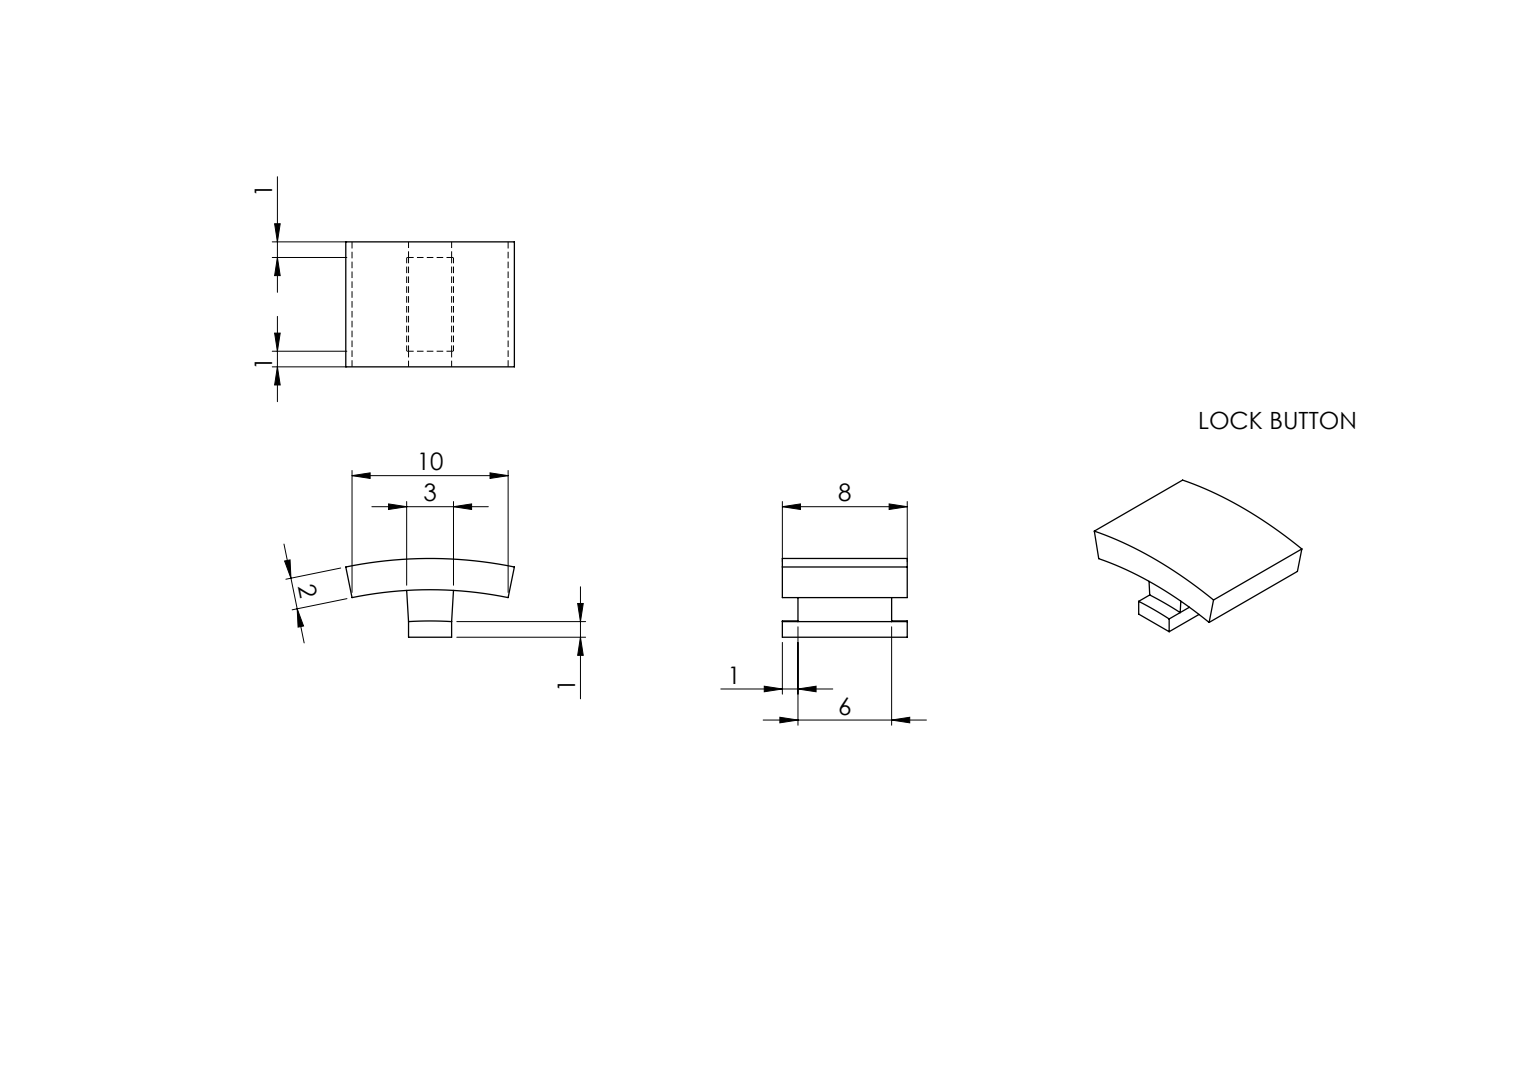
ISO-10303-21;
HEADER;
FILE_DESCRIPTION (('STEP AP214'),
    '1' );
FILE_NAME ('Lock Button.step',
    '2026-10-23T14:45:25',
    ( '' ),
    ( '' ),
    'SwSTEP 2.0',
    'SolidWorks 2026',
    '' );
FILE_SCHEMA (( 'AUTOMOTIVE_DESIGN' ));
ENDSEC;

DATA;
#2=DIRECTION ( 'NONE',  ( -1.000000000000000000, 0.000000000000000000, 0.000000000000000000 ) ) ;
#23=EDGE_CURVE ( 'NONE', #5658, #4842, #4898, .T. ) ;
#26=FILL_AREA_STYLE ('',( #3055 ) ) ;
#34=DIRECTION ( 'NONE',  ( 0.000000000000000000, 0.000000000000000000, -1.000000000000000000 ) ) ;
#40=CIRCLE ( 'NONE', #4910, 25.00000000000000000 ) ;
#55=CARTESIAN_POINT ( 'NONE',  ( 1.380000000000002336, 22.95856267278071172, 12.00000000000000000 ) ) ;
#65=ORIENTED_EDGE ( 'NONE', *, *, #4214, .F. ) ;
#72=VECTOR ( 'NONE', #3186, 1000.000000000000000 ) ;
#83=( NAMED_UNIT ( * ) SI_UNIT ( $, .STERADIAN. ) SOLID_ANGLE_UNIT ( ) );
#84=CARTESIAN_POINT ( 'NONE',  ( 1.380000000000002558, 22.95856267278071527, 1.371299631966804711 ) ) ;
#116=DIRECTION ( 'NONE',  ( 2.385244779468107388E-15, 1.000000000000000000, 0.000000000000000000 ) ) ;
#117=ORIENTED_EDGE ( 'NONE', *, *, #2522, .T. ) ;
#136=PLANE ( 'NONE',  #3174 ) ;
#139=ORIENTED_EDGE ( 'NONE', *, *, #5614, .T. ) ;
#142=LINE ( 'NONE', #1986, #246 ) ;
#143=SHAPE_REPRESENTATION ( 'Lock Button', ( #1336 ), #3242 ) ;
#175=DIRECTION ( 'NONE',  ( -0.000000000000000000, -0.000000000000000000, 1.000000000000000000 ) ) ;
#176=CARTESIAN_POINT ( 'NONE',  ( 1.380000000000002558, 22.95856267278071527, 11.00000000000000000 ) ) ;
#185=FACE_OUTER_BOUND ( 'NONE', #2391, .T. ) ;
#203=LINE ( 'NONE', #3710, #3455 ) ;
#213=DIRECTION ( 'NONE',  ( 0.000000000000000000, 0.000000000000000000, -1.000000000000000000 ) ) ;
#219=AXIS2_PLACEMENT_3D ( 'NONE', #5135, #3840, #5044 ) ;
#220=ORIENTED_EDGE ( 'NONE', *, *, #4170, .T. ) ;
#230=CARTESIAN_POINT ( 'NONE',  ( 1.380000000000002558, 22.95856267278071527, 11.00000000000000000 ) ) ;
#246=VECTOR ( 'NONE', #2299, 1000.000000000000000 ) ;
#267=EDGE_CURVE ( 'NONE', #1755, #5130, #3687, .T. ) ;
#278=FACE_OUTER_BOUND ( 'NONE', #3102, .T. ) ;
#283=CARTESIAN_POINT ( 'NONE',  ( 0.000000000000000000, 0.000000000000000000, 0.000000000000000000 ) ) ;
#295=DIRECTION ( 'NONE',  ( -0.2000000000000000111, 0.9797958971132711969, 0.000000000000000000 ) ) ;
#302=PLANE ( 'NONE',  #1328 ) ;
#303=VECTOR ( 'NONE', #5105, 1000.000000000000000 ) ;
#316=PLANE ( 'NONE',  #4655 ) ;
#324=DIRECTION ( 'NONE',  ( -0.9797958971132711969, 0.2000000000000004552, 0.000000000000000000 ) ) ;
#326=LINE ( 'NONE', #2542, #614 ) ;
#333=ORIENTED_EDGE ( 'NONE', *, *, #340, .F. ) ;
#340=EDGE_CURVE ( 'NONE', #1755, #3088, #1648, .T. ) ;
#346=DIRECTION ( 'NONE',  ( 0.000000000000000000, 0.000000000000000000, -1.000000000000000000 ) ) ;
#357=DIRECTION ( 'NONE',  ( -1.000000000000000000, 0.000000000000000000, 0.000000000000000000 ) ) ;
#364=EDGE_CURVE ( 'NONE', #1139, #4301, #2266, .T. ) ;
#373=DIRECTION ( 'NONE',  ( -0.000000000000000000, -0.000000000000000000, 1.000000000000000000 ) ) ;
#378=DIRECTION ( 'NONE',  ( -0.2000000000000004552, -0.9797958971132711969, 0.000000000000000000 ) ) ;
#389=PRODUCT_DEFINITION_FORMATION_WITH_SPECIFIED_SOURCE ( 'ANY', '', #4589, .NOT_KNOWN. ) ;
#398=ADVANCED_FACE ( 'NONE', ( #2533 ), #316, .T. ) ;
#413=DIRECTION ( 'NONE',  ( 0.000000000000000000, 0.000000000000000000, -1.000000000000000000 ) ) ;
#417=AXIS2_PLACEMENT_3D ( 'NONE', #1217, #3404, #5182 ) ;
#426=AXIS2_PLACEMENT_3D ( 'NONE', #2854, #1529, #4607 ) ;
#431=( NAMED_UNIT ( * ) SI_UNIT ( $, .STERADIAN. ) SOLID_ANGLE_UNIT ( ) );
#435=CARTESIAN_POINT ( 'NONE',  ( 0.000000000000000000, 21.95856267278071527, 4.000000000000000000 ) ) ;
#438=VECTOR ( 'NONE', #2, 1000.000000000000000 ) ;
#465=VERTEX_POINT ( 'NONE', #2969 ) ;
#474=CARTESIAN_POINT ( 'NONE',  ( 1.500000000000003109, 24.95495942693557012, 11.00000000000000000 ) ) ;
#486=DIRECTION ( 'NONE',  ( 1.000000000000000000, -2.385244779468107388E-15, 0.000000000000000000 ) ) ;
#489=CIRCLE ( 'NONE', #219, 25.00000000000000355 ) ;
#491=LINE ( 'NONE', #4006, #5389 ) ;
#496=AXIS2_PLACEMENT_3D ( 'NONE', #3912, #833, #2699 ) ;
#500=EDGE_CURVE ( 'NONE', #1550, #3604, #3484, .T. ) ;
#509=ADVANCED_FACE ( 'NONE', ( #3541 ), #2245, .F. ) ;
#526=DIRECTION ( 'NONE',  ( 1.000000000000000000, 0.000000000000000000, 0.000000000000000000 ) ) ;
#542=DIRECTION ( 'NONE',  ( -1.000000000000000000, 0.000000000000000000, 0.000000000000000000 ) ) ;
#544=ORIENTED_EDGE ( 'NONE', *, *, #3049, .T. ) ;
#546=CARTESIAN_POINT ( 'NONE',  ( -5.399999999999998579, 26.45448922205832787, 12.00000000000000000 ) ) ;
#563=ORIENTED_EDGE ( 'NONE', *, *, #3394, .F. ) ;
#565=FACE_OUTER_BOUND ( 'NONE', #5136, .T. ) ;
#574=CARTESIAN_POINT ( 'NONE',  ( 0.000000000000000000, 0.000000000000000000, 12.00000000000000000 ) ) ;
#575=UNCERTAINTY_MEASURE_WITH_UNIT (LENGTH_MEASURE( 1.000000000000000082E-05 ), #4830, 'distance_accuracy_value', 'NONE');
#607=AXIS2_PLACEMENT_3D ( 'NONE', #2707, #486, #5329 ) ;
#612=VECTOR ( 'NONE', #526, 1000.000000000000000 ) ;
#614=VECTOR ( 'NONE', #4305, 1000.000000000000000 ) ;
#620=PLANE ( 'NONE',  #2643 ) ;
#672=LINE ( 'NONE', #2886, #5086 ) ;
#682=EDGE_LOOP ( 'NONE', ( #5307, #2020, #1568, #4865 ) ) ;
#686=CARTESIAN_POINT ( 'NONE',  ( -4.999999999999998224, 24.49489742783178414, 12.00000000000000000 ) ) ;
#694=ADVANCED_BREP_SHAPE_REPRESENTATION ( '', ( #4492, #1336 ), #3242 ) ;
#709=CARTESIAN_POINT ( 'NONE',  ( 0.000000000000000000, 0.000000000000000000, 11.00000000000000000 ) ) ;
#731=CARTESIAN_POINT ( 'NONE',  ( 5.000000000000001776, 24.49489742783178414, 4.000000000000000000 ) ) ;
#733=DIRECTION ( 'NONE',  ( -1.000000000000000000, 0.000000000000000000, 0.000000000000000000 ) ) ;
#739=ORIENTED_EDGE ( 'NONE', *, *, #1001, .T. ) ;
#748=EDGE_CURVE ( 'NONE', #4516, #5521, #2767, .T. ) ;
#752=EDGE_CURVE ( 'NONE', #5339, #4697, #142, .T. ) ;
#758=CARTESIAN_POINT ( 'NONE',  ( 5.000000000000001776, 24.49489742783178414, 12.00000000000000000 ) ) ;
#759=COLOUR_RGB ( '',0.8941176470588234615, 0.8941176470588234615, 0.8941176470588234615 ) ;
#760=VERTEX_POINT ( 'NONE', #4973 ) ;
#766=ORIENTED_EDGE ( 'NONE', *, *, #23, .T. ) ;
#784=DIRECTION ( 'NONE',  ( -1.000000000000000000, 0.000000000000000000, -0.000000000000000000 ) ) ;
#790=DIRECTION ( 'NONE',  ( -1.000000000000000000, 0.000000000000000000, 0.000000000000000000 ) ) ;
#793=PRODUCT_DEFINITION_CONTEXT ( 'detailed design', #822, 'design' ) ;
#794=VECTOR ( 'NONE', #5528, 1000.000000000000000 ) ;
#798=VECTOR ( 'NONE', #1497, 1000.000000000000114 ) ;
#819=LINE ( 'NONE', #5620, #3283 ) ;
#822=APPLICATION_CONTEXT ( 'automotive_design' ) ;
#833=DIRECTION ( 'NONE',  ( 0.000000000000000000, 0.000000000000000000, -1.000000000000000000 ) ) ;
#841=VERTEX_POINT ( 'NONE', #4160 ) ;
#847=DIRECTION ( 'NONE',  ( -1.000000000000000000, 0.000000000000000000, -0.000000000000000000 ) ) ;
#855=PRODUCT_CONTEXT ( 'NONE', #5414, 'mechanical' ) ;
#880=ORIENTED_EDGE ( 'NONE', *, *, #4681, .T. ) ;
#884=SHAPE_DEFINITION_REPRESENTATION ( #3763, #143 ) ;
#918=( NAMED_UNIT ( * ) PLANE_ANGLE_UNIT ( ) SI_UNIT ( $, .RADIAN. ) );
#946=( LENGTH_UNIT ( ) NAMED_UNIT ( * ) SI_UNIT ( .MILLI., .METRE. ) );
#955=DIRECTION ( 'NONE',  ( -0.000000000000000000, -0.000000000000000000, 1.000000000000000000 ) ) ;
#957=CARTESIAN_POINT ( 'NONE',  ( 0.000000000000000000, 21.95856267278071527, 12.00000000000000000 ) ) ;
#960=VECTOR ( 'NONE', #1765, 999.9999999999998863 ) ;
#977=CIRCLE ( 'NONE', #3188, 23.00000000000000000 ) ;
#980=PLANE ( 'NONE',  #3743 ) ;
#982=DIRECTION ( 'NONE',  ( 0.000000000000000000, 0.000000000000000000, -1.000000000000000000 ) ) ;
#984=VECTOR ( 'NONE', #3012, 1000.000000000000000 ) ;
#1001=EDGE_CURVE ( 'NONE', #4842, #1005, #1915, .T. ) ;
#1005=VERTEX_POINT ( 'NONE', #2808 ) ;
#1008=ADVANCED_FACE ( 'NONE', ( #4558 ), #620, .T. ) ;
#1034=CYLINDRICAL_SURFACE ( 'NONE', #426, 23.00000000000000000 ) ;
#1045=DIRECTION ( 'NONE',  ( 0.000000000000000000, 0.000000000000000000, -1.000000000000000000 ) ) ;
#1051=ORIENTED_EDGE ( 'NONE', *, *, #3485, .T. ) ;
#1055=CARTESIAN_POINT ( 'NONE',  ( 0.000000000000000000, 0.000000000000000000, 15.94994774640597512 ) ) ;
#1065=DIRECTION ( 'NONE',  ( -1.000000000000000000, 0.000000000000000000, 0.000000000000000000 ) ) ;
#1068=ORIENTED_EDGE ( 'NONE', *, *, #1175, .F. ) ;
#1083=EDGE_CURVE ( 'NONE', #3693, #5521, #326, .T. ) ;
#1097=ORIENTED_EDGE ( 'NONE', *, *, #1110, .F. ) ;
#1110=EDGE_CURVE ( 'NONE', #3088, #5521, #1262, .T. ) ;
#1123=CARTESIAN_POINT ( 'NONE',  ( -5.399999999999998579, 26.45448922205832787, 4.000000000000000000 ) ) ;
#1139=VERTEX_POINT ( 'NONE', #5568 ) ;
#1152=AXIS2_PLACEMENT_3D ( 'NONE', #4637, #2913, #3802 ) ;
#1157=DIRECTION ( 'NONE',  ( 1.000000000000000000, 0.000000000000000000, 0.000000000000000000 ) ) ;
#1160=EDGE_CURVE ( 'NONE', #3604, #1139, #819, .T. ) ;
#1175=EDGE_CURVE ( 'NONE', #3721, #1005, #1198, .T. ) ;
#1187=ORIENTED_EDGE ( 'NONE', *, *, #3561, .T. ) ;
#1198=LINE ( 'NONE', #1680, #984 ) ;
#1203=EDGE_CURVE ( 'NONE', #4044, #4516, #2600, .T. ) ;
#1217=CARTESIAN_POINT ( 'NONE',  ( 0.000000000000000000, 0.000000000000000000, 24.08672805191341482 ) ) ;
#1228=ORIENTED_EDGE ( 'NONE', *, *, #2292, .F. ) ;
#1235=CIRCLE ( 'NONE', #5096, 23.00000000000000000 ) ;
#1245=EDGE_CURVE ( 'NONE', #5361, #1550, #5253, .T. ) ;
#1246=PLANE ( 'NONE',  #4536 ) ;
#1262=CIRCLE ( 'NONE', #1808, 25.00000000000000000 ) ;
#1277=ADVANCED_FACE ( 'NONE', ( #4801 ), #980, .F. ) ;
#1290=ORIENTED_EDGE ( 'NONE', *, *, #4170, .F. ) ;
#1306=CARTESIAN_POINT ( 'NONE',  ( -1.500000000000000888, 24.95495942693557012, 11.00000000000000000 ) ) ;
#1308=CARTESIAN_POINT ( 'NONE',  ( -5.399999999999998579, 26.45448922205832787, 12.00000000000000000 ) ) ;
#1319=ORIENTED_EDGE ( 'NONE', *, *, #1160, .F. ) ;
#1321=AXIS2_PLACEMENT_3D ( 'NONE', #84, #4799, #4376 ) ;
#1328=AXIS2_PLACEMENT_3D ( 'NONE', #2036, #2064, #3821 ) ;
#1336=AXIS2_PLACEMENT_3D ( 'NONE', #283, #2997, #5213 ) ;
#1374=ORIENTED_EDGE ( 'NONE', *, *, #340, .T. ) ;
#1382=LINE ( 'NONE', #1649, #3536 ) ;
#1392=ORIENTED_EDGE ( 'NONE', *, *, #2121, .T. ) ;
#1405=EDGE_CURVE ( 'NONE', #1005, #3984, #4403, .T. ) ;
#1408=PLANE ( 'NONE',  #1321 ) ;
#1468=ORIENTED_EDGE ( 'NONE', *, *, #752, .T. ) ;
#1487=DIRECTION ( 'NONE',  ( -1.000000000000000000, 0.000000000000000000, 0.000000000000000000 ) ) ;
#1495=FACE_OUTER_BOUND ( 'NONE', #3746, .T. ) ;
#1496=VERTEX_POINT ( 'NONE', #2353 ) ;
#1497=DIRECTION ( 'NONE',  ( 0.06000000000000008105, -0.9981983770774224274, 0.000000000000000000 ) ) ;
#1504=ORIENTED_EDGE ( 'NONE', *, *, #4283, .F. ) ;
#1513=ORIENTED_EDGE ( 'NONE', *, *, #5599, .T. ) ;
#1515=CIRCLE ( 'NONE', #1152, 23.00000000000000000 ) ;
#1527=CARTESIAN_POINT ( 'NONE',  ( -1.380000000000002558, 21.95856267278071527, 12.00000000000000000 ) ) ;
#1529=DIRECTION ( 'NONE',  ( 0.000000000000000000, 0.000000000000000000, -1.000000000000000000 ) ) ;
#1535=CLOSED_SHELL ( 'NONE', ( #2866, #5174, #4061, #4351, #5113, #4620, #3495, #398, #2220, #509, #5195, #4989, #1008, #3147, #1277, #2437, #5438 ) ) ;
#1539=DIRECTION ( 'NONE',  ( 0.000000000000000000, 0.000000000000000000, -1.000000000000000000 ) ) ;
#1550=VERTEX_POINT ( 'NONE', #546 ) ;
#1559=CARTESIAN_POINT ( 'NONE',  ( 1.380000000000002336, 22.95856267278071172, 15.94994774640597512 ) ) ;
#1568=ORIENTED_EDGE ( 'NONE', *, *, #4598, .T. ) ;
#1586=ORIENTED_EDGE ( 'NONE', *, *, #364, .F. ) ;
#1602=ORIENTED_EDGE ( 'NONE', *, *, #2842, .F. ) ;
#1613=VECTOR ( 'NONE', #378, 999.9999999999998863 ) ;
#1626=LINE ( 'NONE', #758, #1613 ) ;
#1634=EDGE_LOOP ( 'NONE', ( #1374, #3177, #5626, #5423 ) ) ;
#1648=LINE ( 'NONE', #4324, #4111 ) ;
#1649=CARTESIAN_POINT ( 'NONE',  ( 1.380000000000002558, 22.95856267278071527, 5.000000000000000000 ) ) ;
#1672=ORIENTED_EDGE ( 'NONE', *, *, #2121, .F. ) ;
#1680=CARTESIAN_POINT ( 'NONE',  ( 1.380000000000002558, 0.000000000000000000, 4.000000000000000000 ) ) ;
#1702=FACE_OUTER_BOUND ( 'NONE', #3953, .T. ) ;
#1711=DIRECTION ( 'NONE',  ( 0.000000000000000000, 0.000000000000000000, -1.000000000000000000 ) ) ;
#1728=FACE_OUTER_BOUND ( 'NONE', #4142, .T. ) ;
#1738=EDGE_LOOP ( 'NONE', ( #3774, #739, #1068, #5199, #1051, #3753 ) ) ;
#1751=PRESENTATION_STYLE_ASSIGNMENT (( #3596 ) ) ;
#1755=VERTEX_POINT ( 'NONE', #4256 ) ;
#1765=DIRECTION ( 'NONE',  ( 0.06000000000000009492, -0.9981983770774225384, -0.000000000000000000 ) ) ;
#1778=FACE_BOUND ( 'NONE', #1634, .T. ) ;
#1787=CARTESIAN_POINT ( 'NONE',  ( 0.000000000000000000, 0.000000000000000000, 5.000000000000000000 ) ) ;
#1808=AXIS2_PLACEMENT_3D ( 'NONE', #4331, #3039, #357 ) ;
#1847=CARTESIAN_POINT ( 'NONE',  ( -1.380000000000054960, 3.291637795666119257E-15, 12.00000000000000000 ) ) ;
#1849=ORIENTED_EDGE ( 'NONE', *, *, #3485, .F. ) ;
#1863=DIRECTION ( 'NONE',  ( -0.9981983770774224274, -0.06000000000000008105, 0.000000000000000000 ) ) ;
#1915=LINE ( 'NONE', #3238, #2823 ) ;
#1928=DIRECTION ( 'NONE',  ( 0.000000000000000000, 0.000000000000000000, -1.000000000000000000 ) ) ;
#1939=ORIENTED_EDGE ( 'NONE', *, *, #3806, .T. ) ;
#1956=PLANE ( 'NONE',  #4814 ) ;
#1957=CARTESIAN_POINT ( 'NONE',  ( 1.500000000000002887, 24.95495942693556657, 5.000000000000000000 ) ) ;
#1986=CARTESIAN_POINT ( 'NONE',  ( -1.379999999999999893, 22.95856267278071172, 15.94994774640597512 ) ) ;
#1999=CARTESIAN_POINT ( 'NONE',  ( -4.999999999999999112, 24.49489742783178770, 24.08672805191341482 ) ) ;
#2020=ORIENTED_EDGE ( 'NONE', *, *, #267, .F. ) ;
#2036=CARTESIAN_POINT ( 'NONE',  ( 0.000000000000000000, 0.000000000000000000, 12.00000000000000000 ) ) ;
#2064=DIRECTION ( 'NONE',  ( 0.000000000000000000, 0.000000000000000000, -1.000000000000000000 ) ) ;
#2067=VECTOR ( 'NONE', #2237, 1000.000000000000000 ) ;
#2121=EDGE_CURVE ( 'NONE', #841, #1496, #3215, .T. ) ;
#2138=ORIENTED_EDGE ( 'NONE', *, *, #3394, .T. ) ;
#2151=AXIS2_PLACEMENT_3D ( 'NONE', #4670, #2424, #5070 ) ;
#2164=AXIS2_PLACEMENT_3D ( 'NONE', #3290, #3378, #4692 ) ;
#2178=ORIENTED_EDGE ( 'NONE', *, *, #1405, .T. ) ;
#2188=SURFACE_SIDE_STYLE ('',( #5242 ) ) ;
#2199=DIRECTION ( 'NONE',  ( 0.2000000000000004552, 0.9797958971132711969, 0.000000000000000000 ) ) ;
#2206=ORIENTED_EDGE ( 'NONE', *, *, #3504, .F. ) ;
#2220=ADVANCED_FACE ( 'NONE', ( #2505 ), #2940, .T. ) ;
#2227=LINE ( 'NONE', #4362, #960 ) ;
#2237=DIRECTION ( 'NONE',  ( -0.000000000000000000, 1.000000000000000000, 0.000000000000000000 ) ) ;
#2244=ORIENTED_EDGE ( 'NONE', *, *, #1245, .T. ) ;
#2245=PLANE ( 'NONE',  #607 ) ;
#2266=CIRCLE ( 'NONE', #2355, 25.00000000000000355 ) ;
#2284=ORIENTED_EDGE ( 'NONE', *, *, #5599, .F. ) ;
#2292=EDGE_CURVE ( 'NONE', #4697, #4516, #1515, .T. ) ;
#2293=FACE_OUTER_BOUND ( 'NONE', #3783, .T. ) ;
#2296=EDGE_LOOP ( 'NONE', ( #1672, #544, #2339, #5529 ) ) ;
#2299=DIRECTION ( 'NONE',  ( 0.000000000000000000, 0.000000000000000000, -1.000000000000000000 ) ) ;
#2301=UNCERTAINTY_MEASURE_WITH_UNIT (LENGTH_MEASURE( 1.000000000000000082E-05 ), #4064, 'distance_accuracy_value', 'NONE');
#2316=MECHANICAL_DESIGN_GEOMETRIC_PRESENTATION_REPRESENTATION('',(#5073),#2962);
#2323=ORIENTED_EDGE ( 'NONE', *, *, #500, .F. ) ;
#2335=AXIS2_PLACEMENT_3D ( 'NONE', #1055, #2348, #542 ) ;
#2339=ORIENTED_EDGE ( 'NONE', *, *, #4283, .T. ) ;
#2343=VECTOR ( 'NONE', #2199, 999.9999999999998863 ) ;
#2348=DIRECTION ( 'NONE',  ( 0.000000000000000000, 0.000000000000000000, -1.000000000000000000 ) ) ;
#2353=CARTESIAN_POINT ( 'NONE',  ( 5.400000000000002132, 26.45448922205832432, 4.000000000000000000 ) ) ;
#2355=AXIS2_PLACEMENT_3D ( 'NONE', #2564, #4265, #3427 ) ;
#2361=CARTESIAN_POINT ( 'NONE',  ( 0.000000000000000000, 0.000000000000000000, 5.000000000000000000 ) ) ;
#2372=ORIENTED_EDGE ( 'NONE', *, *, #2842, .T. ) ;
#2379=EDGE_CURVE ( 'NONE', #4336, #3693, #1382, .T. ) ;
#2391=EDGE_LOOP ( 'NONE', ( #1097, #3200, #3123, #2758 ) ) ;
#2424=DIRECTION ( 'NONE',  ( 0.000000000000000000, 0.000000000000000000, -1.000000000000000000 ) ) ;
#2437=ADVANCED_FACE ( 'NONE', ( #1702 ), #3166, .T. ) ;
#2447=VECTOR ( 'NONE', #116, 1000.000000000000000 ) ;
#2488=ORIENTED_EDGE ( 'NONE', *, *, #4273, .F. ) ;
#2505=FACE_OUTER_BOUND ( 'NONE', #3224, .T. ) ;
#2516=( GEOMETRIC_REPRESENTATION_CONTEXT ( 3 ) GLOBAL_UNCERTAINTY_ASSIGNED_CONTEXT ( ( #2301 ) ) GLOBAL_UNIT_ASSIGNED_CONTEXT ( ( #4064, #3577, #3148 ) ) REPRESENTATION_CONTEXT ( 'NONE', 'WORKASPACE' ) );
#2522=EDGE_CURVE ( 'NONE', #4842, #4044, #4749, .T. ) ;
#2533=FACE_OUTER_BOUND ( 'NONE', #1738, .T. ) ;
#2542=CARTESIAN_POINT ( 'NONE',  ( 1.500000000000002887, 24.95495942693556302, 1.371299631966804711 ) ) ;
#2548=DIRECTION ( 'NONE',  ( 0.000000000000000000, 0.000000000000000000, -1.000000000000000000 ) ) ;
#2564=CARTESIAN_POINT ( 'NONE',  ( 0.000000000000000000, 0.000000000000000000, 4.000000000000000000 ) ) ;
#2570=CARTESIAN_POINT ( 'NONE',  ( 5.000000000000001776, 24.49489742783178414, 4.000000000000000000 ) ) ;
#2591=EDGE_LOOP ( 'NONE', ( #65, #2244, #3892, #5539 ) ) ;
#2600=LINE ( 'NONE', #2947, #3469 ) ;
#2625=ORIENTED_EDGE ( 'NONE', *, *, #1245, .F. ) ;
#2628=AXIS2_PLACEMENT_3D ( 'NONE', #3037, #324, #5679 ) ;
#2643=AXIS2_PLACEMENT_3D ( 'NONE', #3435, #413, #790 ) ;
#2659=ORIENTED_EDGE ( 'NONE', *, *, #3049, .F. ) ;
#2666=ORIENTED_EDGE ( 'NONE', *, *, #267, .T. ) ;
#2669=UNCERTAINTY_MEASURE_WITH_UNIT (LENGTH_MEASURE( 1.000000000000000082E-05 ), #946, 'distance_accuracy_value', 'NONE');
#2675=FACE_OUTER_BOUND ( 'NONE', #5511, .T. ) ;
#2699=DIRECTION ( 'NONE',  ( -1.000000000000000000, 0.000000000000000000, 0.000000000000000000 ) ) ;
#2706=EDGE_LOOP ( 'NONE', ( #563, #1187, #139, #880 ) ) ;
#2707=CARTESIAN_POINT ( 'NONE',  ( -1.380000000000054960, 3.291637795666119257E-15, 15.94994774640597512 ) ) ;
#2712=LINE ( 'NONE', #1847, #2447 ) ;
#2715=ORIENTED_EDGE ( 'NONE', *, *, #3132, .F. ) ;
#2735=SHAPE_REPRESENTATION_RELATIONSHIP ( 'NONE' , 'NONE' ,  #143, #694 ) ;
#2754=CARTESIAN_POINT ( 'NONE',  ( 5.400000000000002132, 26.45448922205832432, 24.08672805191341482 ) ) ;
#2758=ORIENTED_EDGE ( 'NONE', *, *, #748, .T. ) ;
#2767=LINE ( 'NONE', #230, #5124 ) ;
#2786=ORIENTED_EDGE ( 'NONE', *, *, #1001, .F. ) ;
#2808=CARTESIAN_POINT ( 'NONE',  ( 1.380000000000002558, 21.95856267278071527, 4.000000000000000000 ) ) ;
#2813=VECTOR ( 'NONE', #3975, 1000.000000000000000 ) ;
#2823=VECTOR ( 'NONE', #1045, 1000.000000000000000 ) ;
#2827=FACE_OUTER_BOUND ( 'NONE', #3761, .T. ) ;
#2828=LINE ( 'NONE', #3342, #794 ) ;
#2842=EDGE_CURVE ( 'NONE', #5339, #4044, #3364, .T. ) ;
#2854=CARTESIAN_POINT ( 'NONE',  ( 0.000000000000000000, 0.000000000000000000, 15.94994774640597512 ) ) ;
#2862=PLANE ( 'NONE',  #5201 ) ;
#2863=ORIENTED_EDGE ( 'NONE', *, *, #1175, .T. ) ;
#2866=ADVANCED_FACE ( 'NONE', ( #185 ), #2862, .F. ) ;
#2877=DIRECTION ( 'NONE',  ( 0.06000000000000009492, 0.9981983770774225384, 0.000000000000000000 ) ) ;
#2886=CARTESIAN_POINT ( 'NONE',  ( 5.000000000000001776, 24.49489742783178414, 24.08672805191341482 ) ) ;
#2904=AXIS2_PLACEMENT_3D ( 'NONE', #4644, #3353, #733 ) ;
#2913=DIRECTION ( 'NONE',  ( 0.000000000000000000, 0.000000000000000000, -1.000000000000000000 ) ) ;
#2940=PLANE ( 'NONE',  #2164 ) ;
#2947=CARTESIAN_POINT ( 'NONE',  ( 1.380000000000002336, 22.95856267278071172, 15.94994774640597512 ) ) ;
#2962=( GEOMETRIC_REPRESENTATION_CONTEXT ( 3 ) GLOBAL_UNCERTAINTY_ASSIGNED_CONTEXT ( ( #575 ) ) GLOBAL_UNIT_ASSIGNED_CONTEXT ( ( #4830, #4454, #83 ) ) REPRESENTATION_CONTEXT ( 'NONE', 'WORKASPACE' ) );
#2969=CARTESIAN_POINT ( 'NONE',  ( 5.000000000000001776, 24.49489742783178414, 12.00000000000000000 ) ) ;
#2974=ORIENTED_EDGE ( 'NONE', *, *, #752, .F. ) ;
#2975=PLANE ( 'NONE',  #2628 ) ;
#2997=DIRECTION ( 'NONE',  ( 0.000000000000000000, 0.000000000000000000, 1.000000000000000000 ) ) ;
#3008=ORIENTED_EDGE ( 'NONE', *, *, #3504, .T. ) ;
#3012=DIRECTION ( 'NONE',  ( 0.000000000000000000, -1.000000000000000000, 0.000000000000000000 ) ) ;
#3036=ORIENTED_EDGE ( 'NONE', *, *, #4681, .F. ) ;
#3037=CARTESIAN_POINT ( 'NONE',  ( 5.000000000000001776, 24.49489742783178414, 24.08672805191341482 ) ) ;
#3039=DIRECTION ( 'NONE',  ( 0.000000000000000000, 0.000000000000000000, -1.000000000000000000 ) ) ;
#3049=EDGE_CURVE ( 'NONE', #841, #465, #1626, .T. ) ;
#3055=FILL_AREA_STYLE_COLOUR ( '', #759 ) ;
#3058=CARTESIAN_POINT ( 'NONE',  ( 1.380000000000002336, 22.95856267278071172, 4.000000000000000000 ) ) ;
#3060=ORIENTED_EDGE ( 'NONE', *, *, #4668, .F. ) ;
#3070=CARTESIAN_POINT ( 'NONE',  ( -1.379999999999999893, 22.95856267278071172, 11.00000000000000000 ) ) ;
#3088=VERTEX_POINT ( 'NONE', #1306 ) ;
#3102=EDGE_LOOP ( 'NONE', ( #1513, #2625, #2488, #2659 ) ) ;
#3123=ORIENTED_EDGE ( 'NONE', *, *, #2292, .T. ) ;
#3132=EDGE_CURVE ( 'NONE', #4301, #1496, #5189, .T. ) ;
#3143=DIRECTION ( 'NONE',  ( 0.9797958971132711969, 0.2000000000000000111, 0.000000000000000000 ) ) ;
#3147=ADVANCED_FACE ( 'NONE', ( #3925 ), #2975, .F. ) ;
#3148=( NAMED_UNIT ( * ) SI_UNIT ( $, .STERADIAN. ) SOLID_ANGLE_UNIT ( ) );
#3166=CYLINDRICAL_SURFACE ( 'NONE', #417, 27.00000000000000355 ) ;
#3174=AXIS2_PLACEMENT_3D ( 'NONE', #4054, #1863, #3621 ) ;
#3177=ORIENTED_EDGE ( 'NONE', *, *, #1110, .T. ) ;
#3186=DIRECTION ( 'NONE',  ( 0.000000000000000000, 0.000000000000000000, -1.000000000000000000 ) ) ;
#3188=AXIS2_PLACEMENT_3D ( 'NONE', #2361, #3257, #5008 ) ;
#3196=VECTOR ( 'NONE', #295, 1000.000000000000114 ) ;
#3200=ORIENTED_EDGE ( 'NONE', *, *, #4668, .T. ) ;
#3213=EDGE_LOOP ( 'NONE', ( #220, #2715, #1586, #1319 ) ) ;
#3215=LINE ( 'NONE', #2754, #72 ) ;
#3221=FACE_OUTER_BOUND ( 'NONE', #2706, .T. ) ;
#3224=EDGE_LOOP ( 'NONE', ( #4557, #1939, #4394, #2786 ) ) ;
#3230=ORIENTED_EDGE ( 'NONE', *, *, #3405, .T. ) ;
#3238=CARTESIAN_POINT ( 'NONE',  ( 1.380000000000002558, 21.95856267278071527, 15.94994774640597512 ) ) ;
#3242=( GEOMETRIC_REPRESENTATION_CONTEXT ( 3 ) GLOBAL_UNCERTAINTY_ASSIGNED_CONTEXT ( ( #2669 ) ) GLOBAL_UNIT_ASSIGNED_CONTEXT ( ( #946, #918, #431 ) ) REPRESENTATION_CONTEXT ( 'NONE', 'WORKASPACE' ) );
#3257=DIRECTION ( 'NONE',  ( 0.000000000000000000, 0.000000000000000000, -1.000000000000000000 ) ) ;
#3283=VECTOR ( 'NONE', #4358, 1000.000000000000114 ) ;
#3290=CARTESIAN_POINT ( 'NONE',  ( 0.000000000000000000, 21.95856267278071527, 15.94994774640597512 ) ) ;
#3342=CARTESIAN_POINT ( 'NONE',  ( -1.380000000000054960, 3.291637795666119257E-15, 4.000000000000000000 ) ) ;
#3351=LINE ( 'NONE', #1999, #303 ) ;
#3353=DIRECTION ( 'NONE',  ( 0.000000000000000000, 0.000000000000000000, -1.000000000000000000 ) ) ;
#3364=CIRCLE ( 'NONE', #2904, 23.00000000000000000 ) ;
#3378=DIRECTION ( 'NONE',  ( 0.000000000000000000, -1.000000000000000000, -0.000000000000000000 ) ) ;
#3394=EDGE_CURVE ( 'NONE', #5130, #760, #3631, .T. ) ;
#3404=DIRECTION ( 'NONE',  ( 0.000000000000000000, 0.000000000000000000, -1.000000000000000000 ) ) ;
#3405=EDGE_CURVE ( 'NONE', #5130, #4697, #491, .T. ) ;
#3416=EDGE_CURVE ( 'NONE', #5658, #5339, #2712, .T. ) ;
#3427=DIRECTION ( 'NONE',  ( -1.000000000000000000, 0.000000000000000000, 0.000000000000000000 ) ) ;
#3435=CARTESIAN_POINT ( 'NONE',  ( 0.000000000000000000, 0.000000000000000000, 4.000000000000000000 ) ) ;
#3455=VECTOR ( 'NONE', #4663, 1000.000000000000000 ) ;
#3469=VECTOR ( 'NONE', #1711, 1000.000000000000000 ) ;
#3484=LINE ( 'NONE', #3574, #5486 ) ;
#3485=EDGE_CURVE ( 'NONE', #4336, #4516, #203, .T. ) ;
#3495=ADVANCED_FACE ( 'NONE', ( #1495 ), #1034, .T. ) ;
#3504=EDGE_CURVE ( 'NONE', #760, #3984, #2828, .T. ) ;
#3515=ORIENTED_EDGE ( 'NONE', *, *, #2379, .T. ) ;
#3536=VECTOR ( 'NONE', #3992, 1000.000000000000114 ) ;
#3541=FACE_OUTER_BOUND ( 'NONE', #5315, .T. ) ;
#3547=ORIENTED_EDGE ( 'NONE', *, *, #1083, .T. ) ;
#3548=ORIENTED_EDGE ( 'NONE', *, *, #3416, .F. ) ;
#3561=EDGE_CURVE ( 'NONE', #5130, #4336, #977, .T. ) ;
#3574=CARTESIAN_POINT ( 'NONE',  ( -5.399999999999998579, 26.45448922205832787, 24.08672805191341482 ) ) ;
#3577=( NAMED_UNIT ( * ) PLANE_ANGLE_UNIT ( ) SI_UNIT ( $, .RADIAN. ) );
#3595=CYLINDRICAL_SURFACE ( 'NONE', #2335, 23.00000000000000000 ) ;
#3596=SURFACE_STYLE_USAGE ( .BOTH. , #2188 ) ;
#3599=DIRECTION ( 'NONE',  ( -0.2000000000000000111, 0.9797958971132711969, 0.000000000000000000 ) ) ;
#3604=VERTEX_POINT ( 'NONE', #1123 ) ;
#3621=DIRECTION ( 'NONE',  ( 0.06000000000000008105, -0.9981983770774224274, 0.000000000000000000 ) ) ;
#3631=LINE ( 'NONE', #4435, #2813 ) ;
#3663=ORIENTED_EDGE ( 'NONE', *, *, #1203, .T. ) ;
#3687=LINE ( 'NONE', #5442, #798 ) ;
#3693=VERTEX_POINT ( 'NONE', #1957 ) ;
#3709=CARTESIAN_POINT ( 'NONE',  ( 0.000000000000000000, 0.000000000000000000, 5.000000000000000000 ) ) ;
#3710=CARTESIAN_POINT ( 'NONE',  ( 1.380000000000002558, 22.95856267278071527, 1.371299631966804711 ) ) ;
#3721=VERTEX_POINT ( 'NONE', #3058 ) ;
#3732=CARTESIAN_POINT ( 'NONE',  ( -1.380000000000000115, 22.95856267278071527, 12.00000000000000000 ) ) ;
#3743=AXIS2_PLACEMENT_3D ( 'NONE', #4378, #3143, #3599 ) ;
#3746=EDGE_LOOP ( 'NONE', ( #1228, #2974, #2372, #3663 ) ) ;
#3753=ORIENTED_EDGE ( 'NONE', *, *, #1203, .F. ) ;
#3761=EDGE_LOOP ( 'NONE', ( #2206, #3036, #2863, #2178 ) ) ;
#3763=PRODUCT_DEFINITION_SHAPE ( 'NONE', 'NONE',  #4780 ) ;
#3774=ORIENTED_EDGE ( 'NONE', *, *, #2522, .F. ) ;
#3783=EDGE_LOOP ( 'NONE', ( #333, #2666, #3230, #3060 ) ) ;
#3802=DIRECTION ( 'NONE',  ( -1.000000000000000000, 0.000000000000000000, 0.000000000000000000 ) ) ;
#3806=EDGE_CURVE ( 'NONE', #5658, #3984, #4233, .T. ) ;
#3821=DIRECTION ( 'NONE',  ( -1.000000000000000000, 0.000000000000000000, 0.000000000000000000 ) ) ;
#3824=VECTOR ( 'NONE', #346, 1000.000000000000000 ) ;
#3840=DIRECTION ( 'NONE',  ( -0.000000000000000000, -0.000000000000000000, 1.000000000000000000 ) ) ;
#3858=CARTESIAN_POINT ( 'NONE',  ( -1.380000000000002558, 21.95856267278071527, 15.94994774640597512 ) ) ;
#3867=ORIENTED_EDGE ( 'NONE', *, *, #3806, .F. ) ;
#3892=ORIENTED_EDGE ( 'NONE', *, *, #500, .T. ) ;
#3912=CARTESIAN_POINT ( 'NONE',  ( 0.000000000000000000, 0.000000000000000000, 24.08672805191341482 ) ) ;
#3924=ORIENTED_EDGE ( 'NONE', *, *, #4214, .T. ) ;
#3925=FACE_OUTER_BOUND ( 'NONE', #2296, .T. ) ;
#3949=CARTESIAN_POINT ( 'NONE',  ( 1.380000000000002336, 22.95856267278071172, 5.000000000000000888 ) ) ;
#3953=EDGE_LOOP ( 'NONE', ( #2284, #1392, #1290, #2323 ) ) ;
#3975=DIRECTION ( 'NONE',  ( 0.000000000000000000, 0.000000000000000000, -1.000000000000000000 ) ) ;
#3984=VERTEX_POINT ( 'NONE', #4889 ) ;
#3986=STYLED_ITEM('',(#5737),#4492);
#3992=DIRECTION ( 'NONE',  ( 0.06000000000000008105, 0.9981983770774224274, 0.000000000000000000 ) ) ;
#4006=CARTESIAN_POINT ( 'NONE',  ( -1.380000000000000115, 22.95856267278071527, 1.371299631966804711 ) ) ;
#4044=VERTEX_POINT ( 'NONE', #55 ) ;
#4054=CARTESIAN_POINT ( 'NONE',  ( -1.500000000000000444, 24.95495942693556302, 1.371299631966804711 ) ) ;
#4061=ADVANCED_FACE ( 'NONE', ( #2675 ), #1408, .T. ) ;
#4064=( LENGTH_UNIT ( ) NAMED_UNIT ( * ) SI_UNIT ( .MILLI., .METRE. ) );
#4082=PLANE ( 'NONE',  #5379 ) ;
#4088=CIRCLE ( 'NONE', #5466, 27.00000000000000355 ) ;
#4111=VECTOR ( 'NONE', #373, 1000.000000000000000 ) ;
#4118=ORIENTED_EDGE ( 'NONE', *, *, #3405, .F. ) ;
#4142=EDGE_LOOP ( 'NONE', ( #1504, #4523, #3924, #4704 ) ) ;
#4160=CARTESIAN_POINT ( 'NONE',  ( 5.400000000000002132, 26.45448922205832432, 12.00000000000000000 ) ) ;
#4170=EDGE_CURVE ( 'NONE', #3604, #1496, #5548, .T. ) ;
#4208=DIRECTION ( 'NONE',  ( -1.000000000000000000, -2.664535259100375697E-15, 0.000000000000000000 ) ) ;
#4214=EDGE_CURVE ( 'NONE', #5361, #1139, #3351, .T. ) ;
#4233=LINE ( 'NONE', #3858, #3824 ) ;
#4236=DIRECTION ( 'NONE',  ( 0.000000000000000000, 0.000000000000000000, -1.000000000000000000 ) ) ;
#4256=CARTESIAN_POINT ( 'NONE',  ( -1.500000000000000888, 24.95495942693557012, 5.000000000000000888 ) ) ;
#4265=DIRECTION ( 'NONE',  ( 0.000000000000000000, 0.000000000000000000, -1.000000000000000000 ) ) ;
#4273=EDGE_CURVE ( 'NONE', #465, #5361, #489, .T. ) ;
#4283=EDGE_CURVE ( 'NONE', #465, #4301, #672, .T. ) ;
#4300=FACE_OUTER_BOUND ( 'NONE', #682, .T. ) ;
#4301=VERTEX_POINT ( 'NONE', #731 ) ;
#4305=DIRECTION ( 'NONE',  ( -0.000000000000000000, -0.000000000000000000, 1.000000000000000000 ) ) ;
#4324=CARTESIAN_POINT ( 'NONE',  ( -1.500000000000000444, 24.95495942693556302, 1.371299631966804711 ) ) ;
#4331=CARTESIAN_POINT ( 'NONE',  ( 0.000000000000000000, 0.000000000000000000, 11.00000000000000000 ) ) ;
#4336=VERTEX_POINT ( 'NONE', #3949 ) ;
#4351=ADVANCED_FACE ( 'NONE', ( #4300 ), #1246, .T. ) ;
#4358=DIRECTION ( 'NONE',  ( 0.2000000000000000111, -0.9797958971132711969, -0.000000000000000000 ) ) ;
#4362=CARTESIAN_POINT ( 'NONE',  ( -1.500000000000000444, 24.95495942693556302, 11.00000000000000000 ) ) ;
#4376=DIRECTION ( 'NONE',  ( 0.06000000000000008105, 0.9981983770774224274, 0.000000000000000000 ) ) ;
#4378=CARTESIAN_POINT ( 'NONE',  ( -5.399999999999998579, 26.45448922205832787, 24.08672805191341482 ) ) ;
#4394=ORIENTED_EDGE ( 'NONE', *, *, #1405, .F. ) ;
#4403=LINE ( 'NONE', #435, #438 ) ;
#4435=CARTESIAN_POINT ( 'NONE',  ( -1.379999999999999893, 22.95856267278071172, 15.94994774640597512 ) ) ;
#4452=VECTOR ( 'NONE', #1928, 1000.000000000000000 ) ;
#4454=( NAMED_UNIT ( * ) PLANE_ANGLE_UNIT ( ) SI_UNIT ( $, .RADIAN. ) );
#4492=MANIFOLD_SOLID_BREP ( 'Extrude-Thin2', #1535 ) ;
#4516=VERTEX_POINT ( 'NONE', #176 ) ;
#4523=ORIENTED_EDGE ( 'NONE', *, *, #4273, .T. ) ;
#4536=AXIS2_PLACEMENT_3D ( 'NONE', #1787, #34, #784 ) ;
#4557=ORIENTED_EDGE ( 'NONE', *, *, #23, .F. ) ;
#4558=FACE_OUTER_BOUND ( 'NONE', #3213, .T. ) ;
#4589=PRODUCT ( 'Lock Button', 'Lock Button', '', ( #855 ) ) ;
#4598=EDGE_CURVE ( 'NONE', #1755, #3693, #40, .T. ) ;
#4607=DIRECTION ( 'NONE',  ( -1.000000000000000000, 0.000000000000000000, 0.000000000000000000 ) ) ;
#4620=ADVANCED_FACE ( 'NONE', ( #2827 ), #1956, .T. ) ;
#4637=CARTESIAN_POINT ( 'NONE',  ( 0.000000000000000000, 0.000000000000000000, 11.00000000000000000 ) ) ;
#4644=CARTESIAN_POINT ( 'NONE',  ( 0.000000000000000000, 0.000000000000000000, 12.00000000000000000 ) ) ;
#4655=AXIS2_PLACEMENT_3D ( 'NONE', #5099, #1157, #4236 ) ;
#4663=DIRECTION ( 'NONE',  ( -0.000000000000000000, -0.000000000000000000, 1.000000000000000000 ) ) ;
#4668=EDGE_CURVE ( 'NONE', #3088, #4697, #2227, .T. ) ;
#4670=CARTESIAN_POINT ( 'NONE',  ( 0.000000000000000000, 0.000000000000000000, 4.000000000000000000 ) ) ;
#4681=EDGE_CURVE ( 'NONE', #3721, #760, #1235, .T. ) ;
#4692=DIRECTION ( 'NONE',  ( 0.000000000000000000, 0.000000000000000000, -1.000000000000000000 ) ) ;
#4697=VERTEX_POINT ( 'NONE', #3070 ) ;
#4704=ORIENTED_EDGE ( 'NONE', *, *, #364, .T. ) ;
#4749=LINE ( 'NONE', #5220, #2067 ) ;
#4780=PRODUCT_DEFINITION ( 'UNKNOWN', '', #389, #793 ) ;
#4788=DIRECTION ( 'NONE',  ( -1.000000000000000000, -8.881784197001250746E-15, 0.000000000000000000 ) ) ;
#4799=DIRECTION ( 'NONE',  ( 0.9981983770774224274, -0.06000000000000008105, 0.000000000000000000 ) ) ;
#4801=FACE_OUTER_BOUND ( 'NONE', #2591, .T. ) ;
#4814=AXIS2_PLACEMENT_3D ( 'NONE', #5469, #2548, #847 ) ;
#4830=( LENGTH_UNIT ( ) NAMED_UNIT ( * ) SI_UNIT ( .MILLI., .METRE. ) );
#4842=VERTEX_POINT ( 'NONE', #4861 ) ;
#4861=CARTESIAN_POINT ( 'NONE',  ( 1.380000000000002558, 21.95856267278071527, 12.00000000000000000 ) ) ;
#4865=ORIENTED_EDGE ( 'NONE', *, *, #2379, .F. ) ;
#4889=CARTESIAN_POINT ( 'NONE',  ( -1.380000000000002558, 21.95856267278071527, 4.000000000000000000 ) ) ;
#4898=LINE ( 'NONE', #957, #612 ) ;
#4910=AXIS2_PLACEMENT_3D ( 'NONE', #3709, #5007, #1065 ) ;
#4916=CARTESIAN_POINT ( 'NONE',  ( -1.379999999999999893, 22.95856267278071172, 5.000000000000000888 ) ) ;
#4973=CARTESIAN_POINT ( 'NONE',  ( -1.379999999999999893, 22.95856267278071172, 4.000000000000000000 ) ) ;
#4989=ADVANCED_FACE ( 'NONE', ( #1728, #1778 ), #5294, .F. ) ;
#4996=CARTESIAN_POINT ( 'NONE',  ( 0.000000000000000000, 0.000000000000000000, 12.00000000000000000 ) ) ;
#5007=DIRECTION ( 'NONE',  ( 0.000000000000000000, 0.000000000000000000, -1.000000000000000000 ) ) ;
#5008=DIRECTION ( 'NONE',  ( -1.000000000000000000, 0.000000000000000000, 0.000000000000000000 ) ) ;
#5036=LINE ( 'NONE', #1559, #4452 ) ;
#5044=DIRECTION ( 'NONE',  ( -1.000000000000000000, -2.664535259100375697E-15, 0.000000000000000000 ) ) ;
#5070=DIRECTION ( 'NONE',  ( -1.000000000000000000, 0.000000000000000000, 0.000000000000000000 ) ) ;
#5072=DIRECTION ( 'NONE',  ( -1.000000000000000000, 0.000000000000000000, 0.000000000000000000 ) ) ;
#5073=STYLED_ITEM ( 'NONE', ( #1751 ), #694 ) ;
#5086=VECTOR ( 'NONE', #1539, 1000.000000000000000 ) ;
#5096=AXIS2_PLACEMENT_3D ( 'NONE', #5656, #5312, #4788 ) ;
#5099=CARTESIAN_POINT ( 'NONE',  ( 1.380000000000002558, 0.000000000000000000, 15.94994774640597512 ) ) ;
#5105=DIRECTION ( 'NONE',  ( 0.000000000000000000, 0.000000000000000000, -1.000000000000000000 ) ) ;
#5113=ADVANCED_FACE ( 'NONE', ( #3221 ), #3595, .T. ) ;
#5124=VECTOR ( 'NONE', #2877, 999.9999999999998863 ) ;
#5130=VERTEX_POINT ( 'NONE', #4916 ) ;
#5135=CARTESIAN_POINT ( 'NONE',  ( 0.000000000000000000, 0.000000000000000000, 12.00000000000000000 ) ) ;
#5136=EDGE_LOOP ( 'NONE', ( #766, #117, #1602, #3548 ) ) ;
#5174=ADVANCED_FACE ( 'NONE', ( #2293 ), #136, .T. ) ;
#5178=MECHANICAL_DESIGN_GEOMETRIC_PRESENTATION_REPRESENTATION('',(#3986),#2516);
#5182=DIRECTION ( 'NONE',  ( -1.000000000000000000, 0.000000000000000000, 0.000000000000000000 ) ) ;
#5189=LINE ( 'NONE', #2570, #2343 ) ;
#5195=ADVANCED_FACE ( 'NONE', ( #565 ), #4082, .F. ) ;
#5199=ORIENTED_EDGE ( 'NONE', *, *, #5614, .F. ) ;
#5201=AXIS2_PLACEMENT_3D ( 'NONE', #709, #213, #5072 ) ;
#5213=DIRECTION ( 'NONE',  ( 1.000000000000000000, 0.000000000000000000, 0.000000000000000000 ) ) ;
#5220=CARTESIAN_POINT ( 'NONE',  ( 1.380000000000002558, 0.000000000000000000, 12.00000000000000000 ) ) ;
#5242=SURFACE_STYLE_FILL_AREA ( #26 ) ;
#5253=LINE ( 'NONE', #1308, #3196 ) ;
#5287=ORIENTED_EDGE ( 'NONE', *, *, #3416, .T. ) ;
#5294=CYLINDRICAL_SURFACE ( 'NONE', #496, 25.00000000000000355 ) ;
#5307=ORIENTED_EDGE ( 'NONE', *, *, #3561, .F. ) ;
#5312=DIRECTION ( 'NONE',  ( -0.000000000000000000, -0.000000000000000000, 1.000000000000000000 ) ) ;
#5315=EDGE_LOOP ( 'NONE', ( #3867, #5287, #1468, #4118, #2138, #3008 ) ) ;
#5329=DIRECTION ( 'NONE',  ( 2.385244779468107388E-15, 1.000000000000000000, 0.000000000000000000 ) ) ;
#5339=VERTEX_POINT ( 'NONE', #3732 ) ;
#5361=VERTEX_POINT ( 'NONE', #686 ) ;
#5379=AXIS2_PLACEMENT_3D ( 'NONE', #4996, #5432, #1487 ) ;
#5389=VECTOR ( 'NONE', #955, 1000.000000000000000 ) ;
#5414=APPLICATION_CONTEXT ( 'automotive_design' ) ;
#5423=ORIENTED_EDGE ( 'NONE', *, *, #4598, .F. ) ;
#5432=DIRECTION ( 'NONE',  ( 0.000000000000000000, 0.000000000000000000, -1.000000000000000000 ) ) ;
#5438=ADVANCED_FACE ( 'NONE', ( #278 ), #302, .F. ) ;
#5442=CARTESIAN_POINT ( 'NONE',  ( -1.500000000000000444, 24.95495942693556302, 5.000000000000000000 ) ) ;
#5466=AXIS2_PLACEMENT_3D ( 'NONE', #574, #175, #4208 ) ;
#5469=CARTESIAN_POINT ( 'NONE',  ( 0.000000000000000000, 0.000000000000000000, 4.000000000000000000 ) ) ;
#5486=VECTOR ( 'NONE', #982, 1000.000000000000000 ) ;
#5489=ORIENTED_EDGE ( 'NONE', *, *, #748, .F. ) ;
#5511=EDGE_LOOP ( 'NONE', ( #1849, #3515, #3547, #5489 ) ) ;
#5521=VERTEX_POINT ( 'NONE', #474 ) ;
#5528=DIRECTION ( 'NONE',  ( -2.385244779468107388E-15, -1.000000000000000000, 0.000000000000000000 ) ) ;
#5529=ORIENTED_EDGE ( 'NONE', *, *, #3132, .T. ) ;
#5539=ORIENTED_EDGE ( 'NONE', *, *, #1160, .T. ) ;
#5548=CIRCLE ( 'NONE', #2151, 27.00000000000000355 ) ;
#5568=CARTESIAN_POINT ( 'NONE',  ( -4.999999999999999112, 24.49489742783178770, 4.000000000000000000 ) ) ;
#5599=EDGE_CURVE ( 'NONE', #841, #1550, #4088, .T. ) ;
#5614=EDGE_CURVE ( 'NONE', #4336, #3721, #5036, .T. ) ;
#5620=CARTESIAN_POINT ( 'NONE',  ( -5.399999999999998579, 26.45448922205832787, 4.000000000000000000 ) ) ;
#5626=ORIENTED_EDGE ( 'NONE', *, *, #1083, .F. ) ;
#5656=CARTESIAN_POINT ( 'NONE',  ( 0.000000000000000000, 0.000000000000000000, 4.000000000000000000 ) ) ;
#5658=VERTEX_POINT ( 'NONE', #1527 ) ;
#5679=DIRECTION ( 'NONE',  ( -0.2000000000000004274, -0.9797958971132710859, 0.000000000000000000 ) ) ;
#5731=COLOUR_RGB('Off White',0.89,0.88,0.83);
#5732=FILL_AREA_STYLE_COLOUR('',#5731);
#5733=FILL_AREA_STYLE('',(#5732));
#5734=SURFACE_STYLE_FILL_AREA(#5733);
#5735=SURFACE_SIDE_STYLE('',(#5734));
#5736=SURFACE_STYLE_USAGE(.BOTH.,#5735);
#5737=PRESENTATION_STYLE_ASSIGNMENT((#5736));
ENDSEC;
END-ISO-10303-21;
